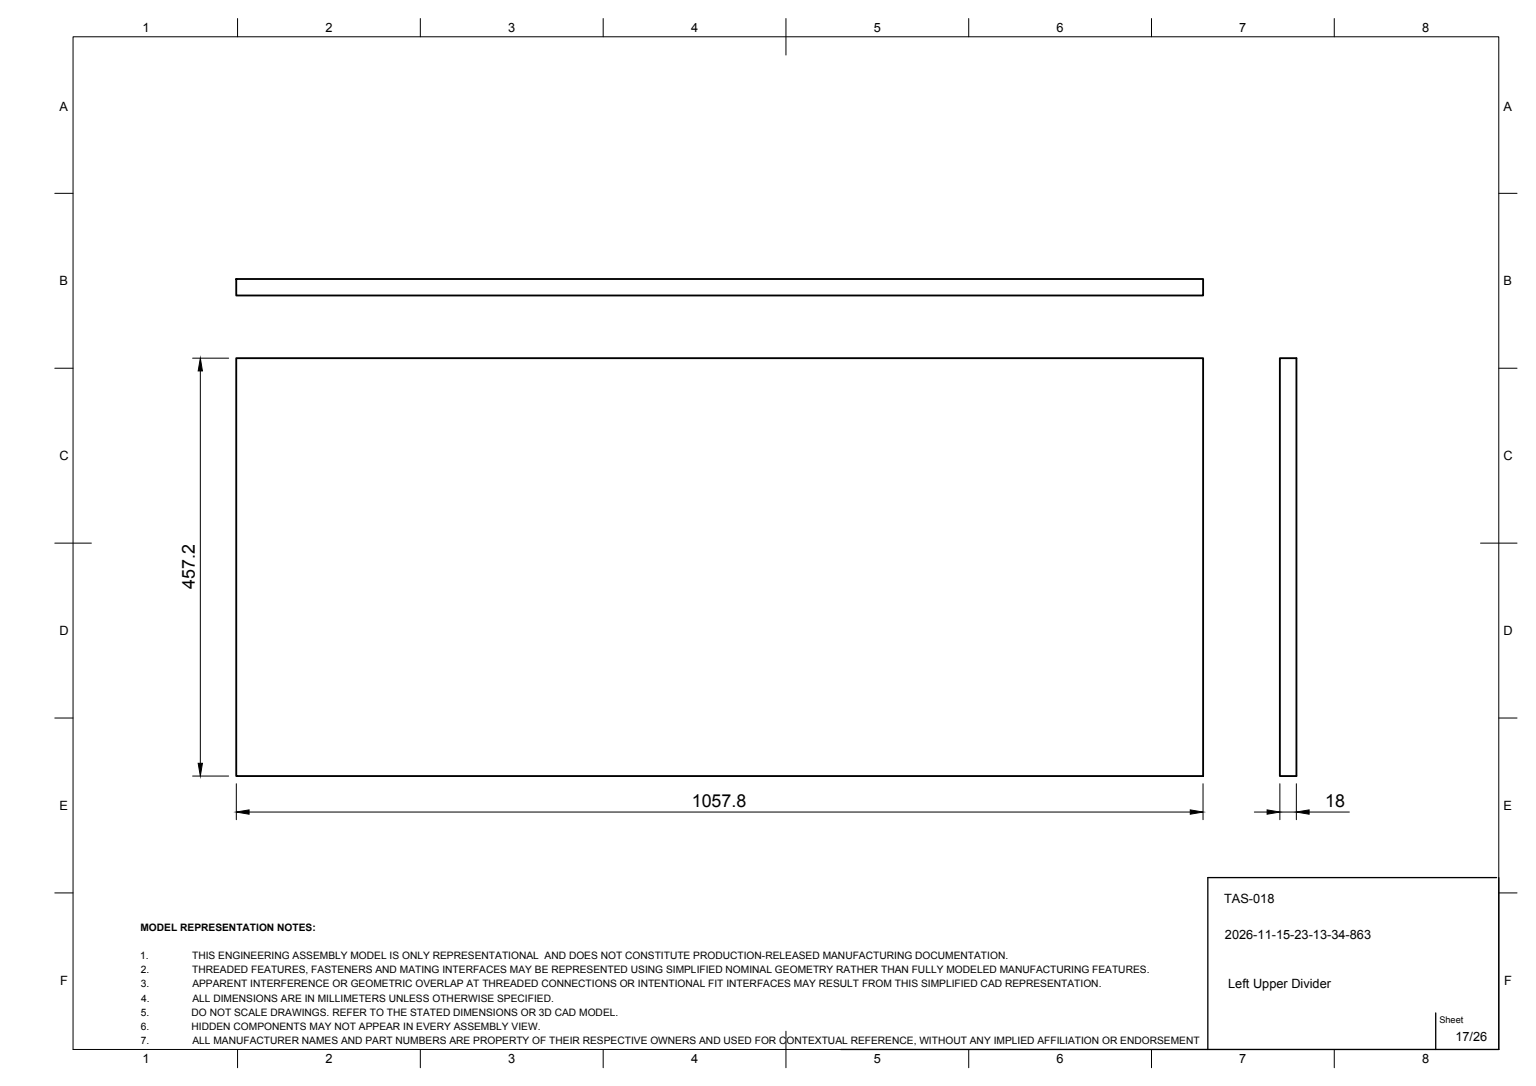
ISO-10303-21;
HEADER;
/* Generated by software containing ST-Developer
 * from STEP Tools, Inc. (www.steptools.com) 
 */

FILE_DESCRIPTION(
/* description */ (''),
/* implementation_level */ '2;1');

FILE_NAME(
/* name */ 'Left Upper Divider.step',
/* time_stamp */ '2026-11-15T15:17:57-08:00',
/* author */ (''),
/* organization */ (''),
/* preprocessor_version */ 'ST-DEVELOPER v20.2',
/* originating_system */ 'Autodesk Translation Framework v15.17.0.0',
/* authorisation */ '');

FILE_SCHEMA (('AUTOMOTIVE_DESIGN { 1 0 10303 214 3 1 1 }'));
ENDSEC;

DATA;
#10=MECHANICAL_DESIGN_GEOMETRIC_PRESENTATION_REPRESENTATION('',(#192),#3723);
#144=SHAPE_REPRESENTATION_RELATIONSHIP('SRR','None',#3825,#168);
#168=ADVANCED_BREP_SHAPE_REPRESENTATION('',(#216),#3714);
#192=STYLED_ITEM('',(#3946),#216);
#216=MANIFOLD_SOLID_BREP('Body1',#2040);
#309=FACE_OUTER_BOUND('',#435,.T.);
#310=FACE_OUTER_BOUND('',#436,.T.);
#311=FACE_OUTER_BOUND('',#437,.T.);
#312=FACE_OUTER_BOUND('',#438,.T.);
#313=FACE_OUTER_BOUND('',#439,.T.);
#314=FACE_OUTER_BOUND('',#440,.T.);
#435=EDGE_LOOP('',(#1635,#1636,#1637,#1638));
#436=EDGE_LOOP('',(#1639,#1640,#1641,#1642));
#437=EDGE_LOOP('',(#1643,#1644,#1645,#1646));
#438=EDGE_LOOP('',(#1647,#1648,#1649,#1650));
#439=EDGE_LOOP('',(#1651,#1652,#1653,#1654));
#440=EDGE_LOOP('',(#1655,#1656,#1657,#1658));
#635=LINE('',#3479,#857);
#636=LINE('',#3481,#858);
#637=LINE('',#3483,#859);
#638=LINE('',#3484,#860);
#639=LINE('',#3487,#861);
#640=LINE('',#3489,#862);
#641=LINE('',#3490,#863);
#642=LINE('',#3493,#864);
#643=LINE('',#3495,#865);
#644=LINE('',#3496,#866);
#645=LINE('',#3498,#867);
#646=LINE('',#3499,#868);
#857=VECTOR('',#2877,41.6456692913386);
#858=VECTOR('',#2878,18.);
#859=VECTOR('',#2879,41.6456692913386);
#860=VECTOR('',#2880,18.);
#861=VECTOR('',#2883,0.708661417322838);
#862=VECTOR('',#2884,0.708661417322838);
#863=VECTOR('',#2885,18.);
#864=VECTOR('',#2888,41.6456692913386);
#865=VECTOR('',#2889,41.6456692913386);
#866=VECTOR('',#2890,18.);
#867=VECTOR('',#2893,0.708661417322836);
#868=VECTOR('',#2894,0.708661417322836);
#1029=VERTEX_POINT('',#3477);
#1030=VERTEX_POINT('',#3478);
#1031=VERTEX_POINT('',#3480);
#1032=VERTEX_POINT('',#3482);
#1033=VERTEX_POINT('',#3486);
#1034=VERTEX_POINT('',#3488);
#1035=VERTEX_POINT('',#3492);
#1036=VERTEX_POINT('',#3494);
#1239=EDGE_CURVE('',#1029,#1030,#635,.T.);
#1240=EDGE_CURVE('',#1029,#1031,#636,.T.);
#1241=EDGE_CURVE('',#1031,#1032,#637,.T.);
#1242=EDGE_CURVE('',#1030,#1032,#638,.T.);
#1243=EDGE_CURVE('',#1030,#1033,#639,.T.);
#1244=EDGE_CURVE('',#1032,#1034,#640,.T.);
#1245=EDGE_CURVE('',#1033,#1034,#641,.T.);
#1246=EDGE_CURVE('',#1033,#1035,#642,.T.);
#1247=EDGE_CURVE('',#1034,#1036,#643,.T.);
#1248=EDGE_CURVE('',#1035,#1036,#644,.T.);
#1249=EDGE_CURVE('',#1035,#1029,#645,.T.);
#1250=EDGE_CURVE('',#1036,#1031,#646,.T.);
#1635=ORIENTED_EDGE('',*,*,#1239,.F.);
#1636=ORIENTED_EDGE('',*,*,#1240,.T.);
#1637=ORIENTED_EDGE('',*,*,#1241,.T.);
#1638=ORIENTED_EDGE('',*,*,#1242,.F.);
#1639=ORIENTED_EDGE('',*,*,#1243,.F.);
#1640=ORIENTED_EDGE('',*,*,#1242,.T.);
#1641=ORIENTED_EDGE('',*,*,#1244,.T.);
#1642=ORIENTED_EDGE('',*,*,#1245,.F.);
#1643=ORIENTED_EDGE('',*,*,#1246,.F.);
#1644=ORIENTED_EDGE('',*,*,#1245,.T.);
#1645=ORIENTED_EDGE('',*,*,#1247,.T.);
#1646=ORIENTED_EDGE('',*,*,#1248,.F.);
#1647=ORIENTED_EDGE('',*,*,#1249,.F.);
#1648=ORIENTED_EDGE('',*,*,#1248,.T.);
#1649=ORIENTED_EDGE('',*,*,#1250,.T.);
#1650=ORIENTED_EDGE('',*,*,#1240,.F.);
#1651=ORIENTED_EDGE('',*,*,#1241,.F.);
#1652=ORIENTED_EDGE('',*,*,#1250,.F.);
#1653=ORIENTED_EDGE('',*,*,#1247,.F.);
#1654=ORIENTED_EDGE('',*,*,#1244,.F.);
#1655=ORIENTED_EDGE('',*,*,#1249,.T.);
#1656=ORIENTED_EDGE('',*,*,#1239,.T.);
#1657=ORIENTED_EDGE('',*,*,#1243,.T.);
#1658=ORIENTED_EDGE('',*,*,#1246,.T.);
#1861=PLANE('',#2421);
#1862=PLANE('',#2422);
#1863=PLANE('',#2423);
#1864=PLANE('',#2424);
#1865=PLANE('',#2425);
#1866=PLANE('',#2426);
#1983=ADVANCED_FACE('',(#309),#1861,.F.);
#1984=ADVANCED_FACE('',(#310),#1862,.F.);
#1985=ADVANCED_FACE('',(#311),#1863,.F.);
#1986=ADVANCED_FACE('',(#312),#1864,.F.);
#1987=ADVANCED_FACE('',(#313),#1865,.F.);
#1988=ADVANCED_FACE('',(#314),#1866,.T.);
#2040=CLOSED_SHELL('',(#1983,#1984,#1985,#1986,#1987,#1988));
#2420=AXIS2_PLACEMENT_3D('',#3475,#2873,#2874);
#2421=AXIS2_PLACEMENT_3D('',#3476,#2875,#2876);
#2422=AXIS2_PLACEMENT_3D('',#3485,#2881,#2882);
#2423=AXIS2_PLACEMENT_3D('',#3491,#2886,#2887);
#2424=AXIS2_PLACEMENT_3D('',#3497,#2891,#2892);
#2425=AXIS2_PLACEMENT_3D('',#3500,#2895,#2896);
#2426=AXIS2_PLACEMENT_3D('',#3501,#2897,#2898);
#2873=DIRECTION('axis',(0.,0.,1.));
#2874=DIRECTION('refdir',(1.,0.,0.));
#2875=DIRECTION('center_axis',(1.,5.24779270478898E-17,0.));
#2876=DIRECTION('ref_axis',(0.,0.,-1.));
#2877=DIRECTION('',(6.71717466212989E-17,-1.,0.));
#2878=DIRECTION('',(0.,0.,-1.));
#2879=DIRECTION('',(6.71717466212989E-17,-1.,0.));
#2880=DIRECTION('',(0.,0.,-1.));
#2881=DIRECTION('center_axis',(0.,1.,0.));
#2882=DIRECTION('ref_axis',(0.,0.,1.));
#2883=DIRECTION('',(1.,0.,0.));
#2884=DIRECTION('',(1.,0.,0.));
#2885=DIRECTION('',(0.,0.,-1.));
#2886=DIRECTION('center_axis',(-1.,-1.0495585409578E-16,0.));
#2887=DIRECTION('ref_axis',(0.,0.,1.));
#2888=DIRECTION('',(-1.00757619931948E-16,1.,0.));
#2889=DIRECTION('',(-1.00757619931948E-16,1.,0.));
#2890=DIRECTION('',(0.,0.,-1.));
#2891=DIRECTION('center_axis',(0.,-1.,0.));
#2892=DIRECTION('ref_axis',(0.,0.,-1.));
#2893=DIRECTION('',(-1.,0.,0.));
#2894=DIRECTION('',(-1.,0.,0.));
#2895=DIRECTION('center_axis',(0.,0.,1.));
#2896=DIRECTION('ref_axis',(1.,0.,0.));
#2897=DIRECTION('center_axis',(0.,0.,1.));
#2898=DIRECTION('ref_axis',(1.,0.,0.));
#3475=CARTESIAN_POINT('',(0.,0.,0.));
#3476=CARTESIAN_POINT('Origin',(-12.7086614173228,66.6456692913386,60.3603597227694));
#3477=CARTESIAN_POINT('',(-12.7086614173228,66.6456692913386,18.7086614173228));
#3478=CARTESIAN_POINT('',(-12.7086614173228,25.,18.7086614173228));
#3479=CARTESIAN_POINT('',(-12.7086614173228,66.6456692913386,18.7086614173228));
#3480=CARTESIAN_POINT('',(-12.7086614173228,66.6456692913386,0.708661417322834));
#3481=CARTESIAN_POINT('',(-12.7086614173228,66.6456692913386,18.7086614173228));
#3482=CARTESIAN_POINT('',(-12.7086614173228,25.,0.708661417322834));
#3483=CARTESIAN_POINT('',(-12.7086614173228,66.6456692913386,0.708661417322834));
#3484=CARTESIAN_POINT('',(-12.7086614173228,25.,18.7086614173228));
#3485=CARTESIAN_POINT('Origin',(-12.7086614173228,25.,60.3603597227694));
#3486=CARTESIAN_POINT('',(-12.,25.,18.7086614173228));
#3487=CARTESIAN_POINT('',(-12.7086614173228,25.,18.7086614173228));
#3488=CARTESIAN_POINT('',(-12.,25.,0.708661417322834));
#3489=CARTESIAN_POINT('',(-12.7086614173228,25.,0.708661417322834));
#3490=CARTESIAN_POINT('',(-12.,25.,18.7086614173228));
#3491=CARTESIAN_POINT('Origin',(-12.,66.6456692913386,60.3603597227694));
#3492=CARTESIAN_POINT('',(-12.,66.6456692913386,18.7086614173228));
#3493=CARTESIAN_POINT('',(-12.,25.,18.7086614173228));
#3494=CARTESIAN_POINT('',(-12.,66.6456692913386,0.708661417322834));
#3495=CARTESIAN_POINT('',(-12.,25.,0.708661417322834));
#3496=CARTESIAN_POINT('',(-12.,66.6456692913386,18.7086614173228));
#3497=CARTESIAN_POINT('Origin',(-12.7086614173228,66.6456692913386,60.3603597227694));
#3498=CARTESIAN_POINT('',(-12.,66.6456692913386,18.7086614173228));
#3499=CARTESIAN_POINT('',(-12.,66.6456692913386,0.708661417322834));
#3500=CARTESIAN_POINT('Origin',(0.,0.,0.708661417322834));
#3501=CARTESIAN_POINT('Origin',(0.,0.,18.7086614173228));
#3687=UNCERTAINTY_MEASURE_WITH_UNIT(LENGTH_MEASURE(0.000393700787401575),
#3725,'DISTANCE_ACCURACY_VALUE',
'Maximum model space distance between geometric entities at asserted c
onnectivities');
#3696=UNCERTAINTY_MEASURE_WITH_UNIT(LENGTH_MEASURE(0.000393700787401575),
#3725,'DISTANCE_ACCURACY_VALUE',
'Maximum model space distance between geometric entities at asserted c
onnectivities');
#3714=(
GEOMETRIC_REPRESENTATION_CONTEXT(3)
GLOBAL_UNCERTAINTY_ASSIGNED_CONTEXT((#3687))
GLOBAL_UNIT_ASSIGNED_CONTEXT((#3725,#3729,#3730))
REPRESENTATION_CONTEXT('','3D')
);
#3723=(
GEOMETRIC_REPRESENTATION_CONTEXT(3)
GLOBAL_UNCERTAINTY_ASSIGNED_CONTEXT((#3696))
GLOBAL_UNIT_ASSIGNED_CONTEXT((#3725,#3729,#3730))
REPRESENTATION_CONTEXT('','3D')
);
#3724=DIMENSIONAL_EXPONENTS(1.,0.,0.,0.,0.,0.,0.);
#3725=(
CONVERSION_BASED_UNIT('inch',#3728)
LENGTH_UNIT()
NAMED_UNIT(#3724)
);
#3726=(
LENGTH_UNIT()
NAMED_UNIT(*)
SI_UNIT(.MILLI.,.METRE.)
);
#3728=LENGTH_MEASURE_WITH_UNIT(LENGTH_MEASURE(25.4),#3726);
#3729=(
NAMED_UNIT(*)
PLANE_ANGLE_UNIT()
SI_UNIT($,.RADIAN.)
);
#3730=(
NAMED_UNIT(*)
SI_UNIT($,.STERADIAN.)
SOLID_ANGLE_UNIT()
);
#3748=SHAPE_DEFINITION_REPRESENTATION(#3775,#3825);
#3775=PRODUCT_DEFINITION_SHAPE('',$,#3852);
#3825=SHAPE_REPRESENTATION('',(#2420),#3714);
#3834=PRODUCT_DEFINITION_CONTEXT('part definition',#3914,'design');
#3852=PRODUCT_DEFINITION('2026-11-15-23-13-34-863','Left Upper Divider',
#3878,#3834);
#3878=PRODUCT_DEFINITION_FORMATION('',$,#3933);
#3914=APPLICATION_CONTEXT(
'Core Data for Automotive Mechanical Design Process');
#3915=PRODUCT_CONTEXT('part definition',#3914,'mechanical');
#3933=PRODUCT('2026-11-15-23-13-34-863','Left Upper Divider',$,(#3915));
#3946=PRESENTATION_STYLE_ASSIGNMENT((#3954));
#3954=SURFACE_STYLE_USAGE(.BOTH.,#3962);
#3962=SURFACE_SIDE_STYLE('',(#3970));
#3970=SURFACE_STYLE_FILL_AREA(#3978);
#3978=FILL_AREA_STYLE('Gray',(#3986));
#3986=FILL_AREA_STYLE_COLOUR('Gray',#3994);
#3994=COLOUR_RGB('Gray',0.501960784313725,0.501960784313725,0.501960784313725);
ENDSEC;
END-ISO-10303-21;
